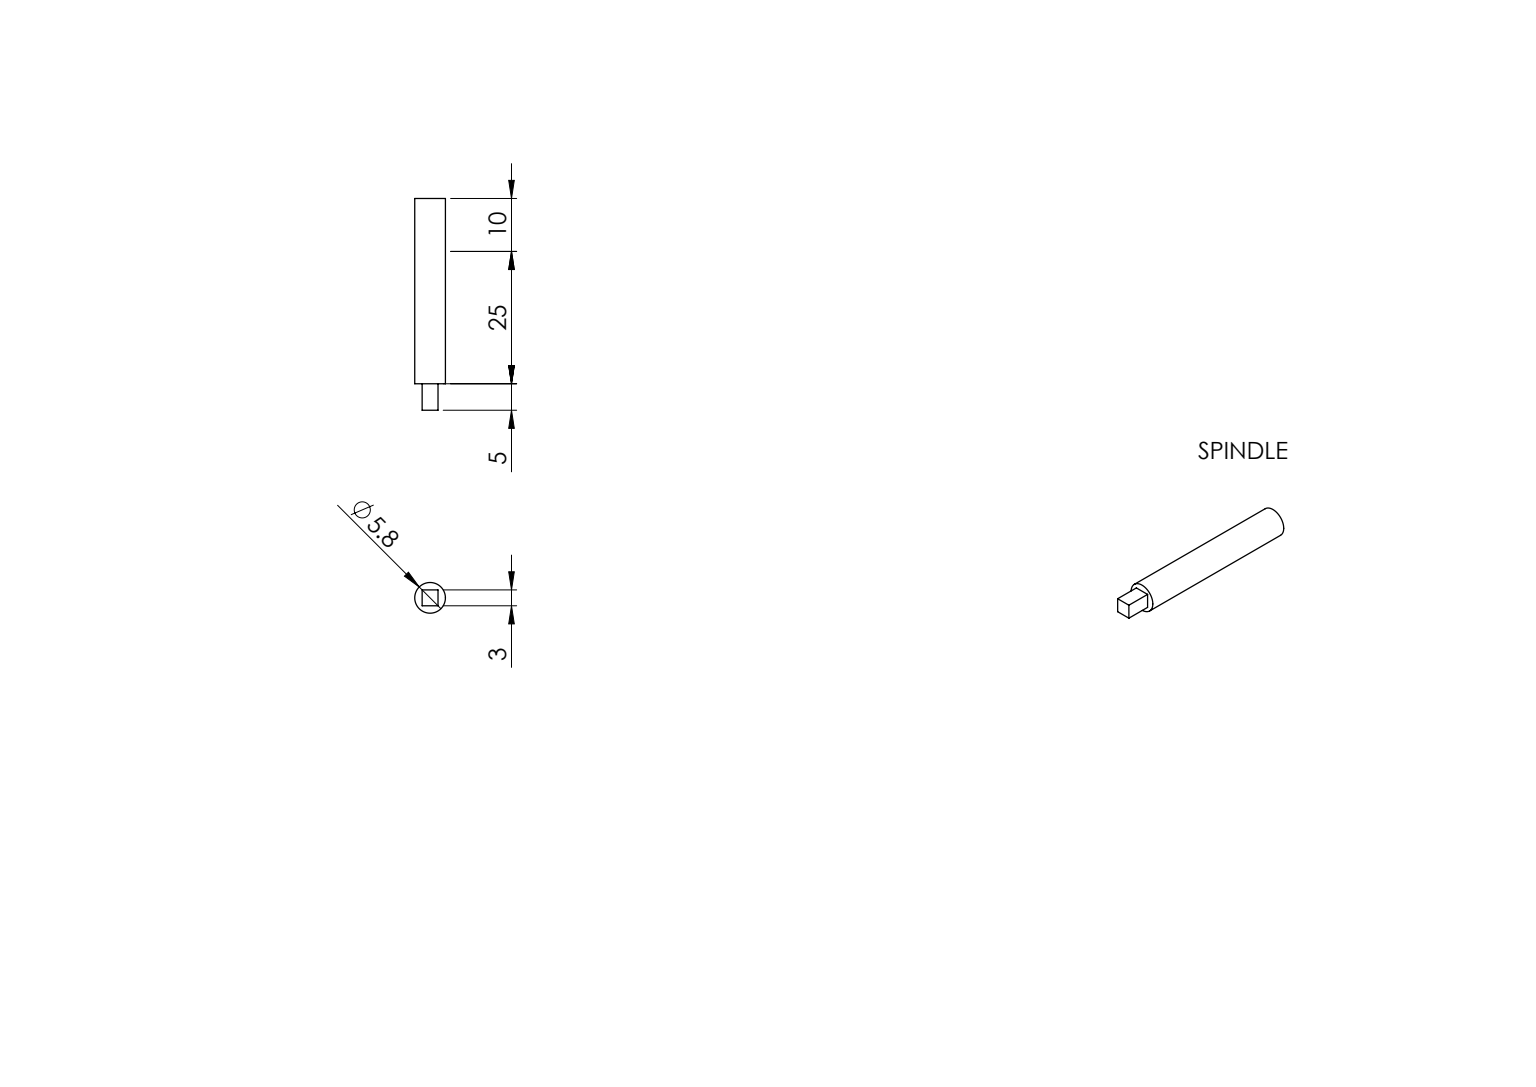
ISO-10303-21;
HEADER;
FILE_DESCRIPTION (('STEP AP214'),
    '1' );
FILE_NAME ('spindle.step',
    '2026-10-26T12:50:16',
    ( '' ),
    ( '' ),
    'SwSTEP 2.0',
    'SolidWorks 2026',
    '' );
FILE_SCHEMA (( 'AUTOMOTIVE_DESIGN' ));
ENDSEC;

DATA;
#229=PRODUCT_DEFINITION ( 'UNKNOWN', '', #18569, #2861 ) ;
#231=( LENGTH_UNIT ( ) NAMED_UNIT ( * ) SI_UNIT ( .MILLI., .METRE. ) );
#248=CARTESIAN_POINT ( 'NONE',  ( -2.899999999999996358, -8.999999999999992895, 25.00000000000000000 ) ) ;
#508=AXIS2_PLACEMENT_3D ( 'NONE', #23574, #21601, #11656 ) ;
#536=DIRECTION ( 'NONE',  ( -0.000000000000000000, -0.000000000000000000, -1.000000000000000000 ) ) ;
#569=( LENGTH_UNIT ( ) NAMED_UNIT ( * ) SI_UNIT ( .MILLI., .METRE. ) );
#621=CARTESIAN_POINT ( 'NONE',  ( 1.500000000000001776, -10.49999999999999289, 25.00000000000000000 ) ) ;
#636=PLANE ( 'NONE',  #20950 ) ;
#809=EDGE_CURVE ( 'NONE', #24918, #4288, #17286, .T. ) ;
#1026=ORIENTED_EDGE ( 'NONE', *, *, #13707, .T. ) ;
#1169=EDGE_CURVE ( 'NONE', #4288, #22996, #9088, .T. ) ;
#1252=PRODUCT_CONTEXT ( 'NONE', #12277, 'mechanical' ) ;
#1277=VERTEX_POINT ( 'NONE', #21768 ) ;
#1291=LINE ( 'NONE', #5217, #20952 ) ;
#1606=CARTESIAN_POINT ( 'NONE',  ( 2.900000000000003464, -8.999999999999992895, 25.00000000000000000 ) ) ;
#1677=CARTESIAN_POINT ( 'NONE',  ( -1.499999999999998224, -10.49999999999999289, 30.00000000000000355 ) ) ;
#2145=VERTEX_POINT ( 'NONE', #9561 ) ;
#2861=PRODUCT_DEFINITION_CONTEXT ( 'detailed design', #19293, 'design' ) ;
#2959=LINE ( 'NONE', #621, #13533 ) ;
#3022=EDGE_CURVE ( 'NONE', #11790, #1277, #20201, .T. ) ;
#3115=EDGE_LOOP ( 'NONE', ( #11167, #14069, #8642, #18079 ) ) ;
#3162=EDGE_CURVE ( 'NONE', #23707, #2145, #4900, .T. ) ;
#3167=ORIENTED_EDGE ( 'NONE', *, *, #10282, .F. ) ;
#3190=CARTESIAN_POINT ( 'NONE',  ( 3.469446951953614189E-15, -8.999999999999992895, -10.00000000000000000 ) ) ;
#3368=VECTOR ( 'NONE', #536, 1000.000000000000000 ) ;
#3395=AXIS2_PLACEMENT_3D ( 'NONE', #1677, #25474, #19072 ) ;
#3413=LINE ( 'NONE', #11515, #13794 ) ;
#3458=DIRECTION ( 'NONE',  ( -0.000000000000000000, -1.000000000000000000, -0.000000000000000000 ) ) ;
#3629=FACE_OUTER_BOUND ( 'NONE', #22399, .T. ) ;
#3707=ORIENTED_EDGE ( 'NONE', *, *, #13635, .T. ) ;
#3902=DIRECTION ( 'NONE',  ( 1.000000000000000000, -2.891205793294678326E-16, 0.000000000000000000 ) ) ;
#3928=CARTESIAN_POINT ( 'NONE',  ( 1.500000000000001776, -7.499999999999993783, 30.00000000000000355 ) ) ;
#3950=ORIENTED_EDGE ( 'NONE', *, *, #25431, .F. ) ;
#4149=PLANE ( 'NONE',  #7144 ) ;
#4224=EDGE_LOOP ( 'NONE', ( #11720, #19596, #3950, #3707 ) ) ;
#4277=FILL_AREA_STYLE ('',( #15786 ) ) ;
#4288=VERTEX_POINT ( 'NONE', #5621 ) ;
#4379=ORIENTED_EDGE ( 'NONE', *, *, #809, .T. ) ;
#4399=( NAMED_UNIT ( * ) PLANE_ANGLE_UNIT ( ) SI_UNIT ( $, .RADIAN. ) );
#4618=FACE_OUTER_BOUND ( 'NONE', #10624, .T. ) ;
#4787=LINE ( 'NONE', #12880, #22930 ) ;
#4900=LINE ( 'NONE', #11041, #15475 ) ;
#5075=ORIENTED_EDGE ( 'NONE', *, *, #1169, .T. ) ;
#5163=CARTESIAN_POINT ( 'NONE',  ( 3.469446951953614189E-15, -8.999999999999992895, 25.00000000000000000 ) ) ;
#5217=CARTESIAN_POINT ( 'NONE',  ( -2.899999999999996358, -8.999999999999992895, -10.00000000000000000 ) ) ;
#5280=DIRECTION ( 'NONE',  ( 1.000000000000000000, 0.000000000000000000, 0.000000000000000000 ) ) ;
#5338=DIRECTION ( 'NONE',  ( 1.000000000000000000, 0.000000000000000000, 0.000000000000000000 ) ) ;
#5380=CIRCLE ( 'NONE', #19982, 2.899999999999999911 ) ;
#5592=ORIENTED_EDGE ( 'NONE', *, *, #21469, .F. ) ;
#5621=CARTESIAN_POINT ( 'NONE',  ( 1.500000000000001776, -10.49999999999999289, 30.00000000000000355 ) ) ;
#5702=ORIENTED_EDGE ( 'NONE', *, *, #15200, .T. ) ;
#5767=EDGE_CURVE ( 'NONE', #2145, #11790, #2959, .T. ) ;
#5867=CARTESIAN_POINT ( 'NONE',  ( 1.500000000000001776, -10.49999999999999289, 30.00000000000000355 ) ) ;
#6229=SURFACE_SIDE_STYLE ('',( #18022 ) ) ;
#6292=ORIENTED_EDGE ( 'NONE', *, *, #21461, .T. ) ;
#6455=ADVANCED_FACE ( 'NONE', ( #17049 ), #17319, .F. ) ;
#6562=CARTESIAN_POINT ( 'NONE',  ( -1.499999999999998224, -7.499999999999992895, 30.00000000000000355 ) ) ;
#6818=ORIENTED_EDGE ( 'NONE', *, *, #18931, .F. ) ;
#6974=ADVANCED_FACE ( 'NONE', ( #22536, #4618 ), #10627, .T. ) ;
#6988=DIRECTION ( 'NONE',  ( 1.000000000000000000, -0.000000000000000000, -0.000000000000000000 ) ) ;
#7144=AXIS2_PLACEMENT_3D ( 'NONE', #12127, #20103, #10166 ) ;
#7146=CIRCLE ( 'NONE', #13012, 2.899999999999999911 ) ;
#7258=LINE ( 'NONE', #11039, #9168 ) ;
#7272=MECHANICAL_DESIGN_GEOMETRIC_PRESENTATION_REPRESENTATION('',(#22295),#10601);
#7376=CYLINDRICAL_SURFACE ( 'NONE', #19185, 2.899999999999999911 ) ;
#7419=CIRCLE ( 'NONE', #7887, 2.899999999999999911 ) ;
#7429=VERTEX_POINT ( 'NONE', #6562 ) ;
#7470=DIRECTION ( 'NONE',  ( 0.000000000000000000, 0.000000000000000000, 1.000000000000000000 ) ) ;
#7576=FACE_OUTER_BOUND ( 'NONE', #14240, .T. ) ;
#7676=( GEOMETRIC_REPRESENTATION_CONTEXT ( 3 ) GLOBAL_UNCERTAINTY_ASSIGNED_CONTEXT ( ( #10971 ) ) GLOBAL_UNIT_ASSIGNED_CONTEXT ( ( #231, #7808, #11863 ) ) REPRESENTATION_CONTEXT ( 'NONE', 'WORKASPACE' ) );
#7808=( NAMED_UNIT ( * ) PLANE_ANGLE_UNIT ( ) SI_UNIT ( $, .RADIAN. ) );
#7887=AXIS2_PLACEMENT_3D ( 'NONE', #5163, #13142, #5280 ) ;
#8126=FACE_OUTER_BOUND ( 'NONE', #17519, .T. ) ;
#8254=EDGE_CURVE ( 'NONE', #22773, #24763, #25592, .T. ) ;
#8445=ORIENTED_EDGE ( 'NONE', *, *, #13635, .F. ) ;
#8476=AXIS2_PLACEMENT_3D ( 'NONE', #22030, #24754, #23873 ) ;
#8531=ADVANCED_FACE ( 'NONE', ( #8126 ), #11787, .T. ) ;
#8642=ORIENTED_EDGE ( 'NONE', *, *, #15200, .F. ) ;
#8785=CARTESIAN_POINT ( 'NONE',  ( -2.899999999999996358, -8.999999999999992895, -10.00000000000000000 ) ) ;
#8843=CARTESIAN_POINT ( 'NONE',  ( 1.500000000000001776, -10.49999999999999289, 30.00000000000000355 ) ) ;
#8998=ORIENTED_EDGE ( 'NONE', *, *, #8254, .T. ) ;
#9061=VERTEX_POINT ( 'NONE', #248 ) ;
#9088=LINE ( 'NONE', #8843, #24740 ) ;
#9168=VECTOR ( 'NONE', #3458, 1000.000000000000000 ) ;
#9334=DIRECTION ( 'NONE',  ( -1.000000000000000000, 2.891205793294678326E-16, 0.000000000000000000 ) ) ;
#9561=CARTESIAN_POINT ( 'NONE',  ( 1.500000000000001776, -10.49999999999999289, 25.00000000000000000 ) ) ;
#9728=CARTESIAN_POINT ( 'NONE',  ( 2.900000000000003464, -8.999999999999992895, -10.00000000000000000 ) ) ;
#9760=ORIENTED_EDGE ( 'NONE', *, *, #21035, .T. ) ;
#9971=LINE ( 'NONE', #9728, #25848 ) ;
#10153=EDGE_CURVE ( 'NONE', #22773, #9061, #1291, .T. ) ;
#10166=DIRECTION ( 'NONE',  ( 0.000000000000000000, 0.000000000000000000, 1.000000000000000000 ) ) ;
#10177=ADVANCED_FACE ( 'NONE', ( #3629 ), #21429, .F. ) ;
#10258=DIRECTION ( 'NONE',  ( -1.000000000000000000, 2.891205793294678326E-16, 0.000000000000000000 ) ) ;
#10282=EDGE_CURVE ( 'NONE', #24763, #22773, #7146, .T. ) ;
#10491=AXIS2_PLACEMENT_3D ( 'NONE', #12859, #25020, #20837 ) ;
#10601=( GEOMETRIC_REPRESENTATION_CONTEXT ( 3 ) GLOBAL_UNCERTAINTY_ASSIGNED_CONTEXT ( ( #17261 ) ) GLOBAL_UNIT_ASSIGNED_CONTEXT ( ( #12116, #4399, #13832 ) ) REPRESENTATION_CONTEXT ( 'NONE', 'WORKASPACE' ) );
#10624=EDGE_LOOP ( 'NONE', ( #5702, #24649 ) ) ;
#10627=PLANE ( 'NONE',  #508 ) ;
#10948=ADVANCED_FACE ( 'NONE', ( #14097 ), #4149, .F. ) ;
#10971=UNCERTAINTY_MEASURE_WITH_UNIT (LENGTH_MEASURE( 1.000000000000000082E-05 ), #231, 'distance_accuracy_value', 'NONE');
#11039=CARTESIAN_POINT ( 'NONE',  ( -1.499999999999998224, -10.49999999999999289, 30.00000000000000355 ) ) ;
#11041=CARTESIAN_POINT ( 'NONE',  ( 1.500000000000001776, -10.49999999999999289, 25.00000000000000000 ) ) ;
#11167=ORIENTED_EDGE ( 'NONE', *, *, #10282, .T. ) ;
#11426=ORIENTED_EDGE ( 'NONE', *, *, #10153, .F. ) ;
#11515=CARTESIAN_POINT ( 'NONE',  ( 1.500000000000001776, -7.499999999999993783, 30.00000000000000355 ) ) ;
#11647=DIRECTION ( 'NONE',  ( 1.000000000000000000, 0.000000000000000000, 0.000000000000000000 ) ) ;
#11656=DIRECTION ( 'NONE',  ( 1.000000000000000000, 0.000000000000000000, -0.000000000000000000 ) ) ;
#11720=ORIENTED_EDGE ( 'NONE', *, *, #3022, .T. ) ;
#11787=CYLINDRICAL_SURFACE ( 'NONE', #18509, 2.899999999999999911 ) ;
#11790=VERTEX_POINT ( 'NONE', #11880 ) ;
#11843=ADVANCED_FACE ( 'NONE', ( #12663 ), #636, .T. ) ;
#11863=( NAMED_UNIT ( * ) SI_UNIT ( $, .STERADIAN. ) SOLID_ANGLE_UNIT ( ) );
#11880=CARTESIAN_POINT ( 'NONE',  ( 1.500000000000001776, -7.499999999999993783, 25.00000000000000000 ) ) ;
#12080=LINE ( 'NONE', #22290, #14598 ) ;
#12116=( LENGTH_UNIT ( ) NAMED_UNIT ( * ) SI_UNIT ( .MILLI., .METRE. ) );
#12126=CARTESIAN_POINT ( 'NONE',  ( 2.900000000000003464, -8.999999999999992895, -10.00000000000000000 ) ) ;
#12127=CARTESIAN_POINT ( 'NONE',  ( 1.500000000000001776, -10.49999999999999289, 30.00000000000000355 ) ) ;
#12252=PRESENTATION_STYLE_ASSIGNMENT (( #14085 ) ) ;
#12261=DIRECTION ( 'NONE',  ( -2.891205793294678326E-16, -1.000000000000000000, 0.000000000000000000 ) ) ;
#12277=APPLICATION_CONTEXT ( 'automotive_design' ) ;
#12376=SHAPE_REPRESENTATION_RELATIONSHIP ( 'NONE' , 'NONE' ,  #13517, #21253 ) ;
#12663=FACE_OUTER_BOUND ( 'NONE', #22952, .T. ) ;
#12750=CARTESIAN_POINT ( 'NONE',  ( 3.469446951953614189E-15, -8.999999999999992895, 25.00000000000000000 ) ) ;
#12859=CARTESIAN_POINT ( 'NONE',  ( 3.469446951953614189E-15, -8.999999999999992895, -10.00000000000000000 ) ) ;
#12880=CARTESIAN_POINT ( 'NONE',  ( -1.499999999999998224, -10.49999999999999289, 25.00000000000000000 ) ) ;
#12983=CLOSED_SHELL ( 'NONE', ( #20116, #8531, #6455, #6974, #10177, #10948, #17461, #24835, #11843 ) ) ;
#13012=AXIS2_PLACEMENT_3D ( 'NONE', #21050, #13462, #5338 ) ;
#13083=VECTOR ( 'NONE', #9334, 1000.000000000000000 ) ;
#13142=DIRECTION ( 'NONE',  ( 0.000000000000000000, 0.000000000000000000, 1.000000000000000000 ) ) ;
#13223=DIRECTION ( 'NONE',  ( 1.000000000000000000, 0.000000000000000000, 0.000000000000000000 ) ) ;
#13271=MANIFOLD_SOLID_BREP ( 'Boss-Extrude2', #12983 ) ;
#13346=CARTESIAN_POINT ( 'NONE',  ( 1.500000000000001776, -10.49999999999999289, 30.00000000000000355 ) ) ;
#13353=CARTESIAN_POINT ( 'NONE',  ( 0.000000000000000000, 0.000000000000000000, 0.000000000000000000 ) ) ;
#13373=ORIENTED_EDGE ( 'NONE', *, *, #19950, .T. ) ;
#13462=DIRECTION ( 'NONE',  ( 0.000000000000000000, 0.000000000000000000, 1.000000000000000000 ) ) ;
#13517=SHAPE_REPRESENTATION ( 'spindle', ( #21036 ), #7676 ) ;
#13533=VECTOR ( 'NONE', #18650, 1000.000000000000000 ) ;
#13635=EDGE_CURVE ( 'NONE', #22996, #11790, #3413, .T. ) ;
#13707=EDGE_CURVE ( 'NONE', #7429, #1277, #22091, .T. ) ;
#13794=VECTOR ( 'NONE', #17539, 1000.000000000000000 ) ;
#13832=( NAMED_UNIT ( * ) SI_UNIT ( $, .STERADIAN. ) SOLID_ANGLE_UNIT ( ) );
#13851=DIRECTION ( 'NONE',  ( -1.000000000000000000, 0.000000000000000000, 0.000000000000000000 ) ) ;
#13856=EDGE_LOOP ( 'NONE', ( #25418, #17554, #23441, #18388 ) ) ;
#14012=CARTESIAN_POINT ( 'NONE',  ( 3.469446951953614189E-15, -8.999999999999992895, -10.00000000000000000 ) ) ;
#14056=DIRECTION ( 'NONE',  ( -0.000000000000000000, -0.000000000000000000, -1.000000000000000000 ) ) ;
#14069=ORIENTED_EDGE ( 'NONE', *, *, #10153, .T. ) ;
#14085=SURFACE_STYLE_USAGE ( .BOTH. , #6229 ) ;
#14097=FACE_OUTER_BOUND ( 'NONE', #19474, .T. ) ;
#14240=EDGE_LOOP ( 'NONE', ( #17690, #8445, #17476, #6292 ) ) ;
#14396=CARTESIAN_POINT ( 'NONE',  ( -1.499999999999998224, -7.499999999999992895, 30.00000000000000355 ) ) ;
#14411=ORIENTED_EDGE ( 'NONE', *, *, #21469, .T. ) ;
#14450=LINE ( 'NONE', #23991, #24620 ) ;
#14555=ORIENTED_EDGE ( 'NONE', *, *, #3162, .T. ) ;
#14598=VECTOR ( 'NONE', #14056, 1000.000000000000000 ) ;
#14661=ORIENTED_EDGE ( 'NONE', *, *, #8254, .F. ) ;
#15200=EDGE_CURVE ( 'NONE', #21831, #9061, #7419, .T. ) ;
#15311=EDGE_CURVE ( 'NONE', #24763, #21831, #9971, .T. ) ;
#15475=VECTOR ( 'NONE', #6988, 1000.000000000000000 ) ;
#15548=DIRECTION ( 'NONE',  ( 0.000000000000000000, 0.000000000000000000, 1.000000000000000000 ) ) ;
#15703=DIRECTION ( 'NONE',  ( 0.000000000000000000, 0.000000000000000000, 1.000000000000000000 ) ) ;
#15741=DIRECTION ( 'NONE',  ( 0.000000000000000000, 0.000000000000000000, 1.000000000000000000 ) ) ;
#15786=FILL_AREA_STYLE_COLOUR ( '', #18551 ) ;
#16121=PRODUCT_DEFINITION_SHAPE ( 'NONE', 'NONE',  #229 ) ;
#16546=VECTOR ( 'NONE', #19219, 1000.000000000000000 ) ;
#16683=DIRECTION ( 'NONE',  ( -0.000000000000000000, -1.000000000000000000, -0.000000000000000000 ) ) ;
#16687=DIRECTION ( 'NONE',  ( 0.000000000000000000, 1.000000000000000000, 0.000000000000000000 ) ) ;
#17049=FACE_OUTER_BOUND ( 'NONE', #24885, .T. ) ;
#17104=AXIS2_PLACEMENT_3D ( 'NONE', #5867, #13851, #19972 ) ;
#17261=UNCERTAINTY_MEASURE_WITH_UNIT (LENGTH_MEASURE( 1.000000000000000082E-05 ), #12116, 'distance_accuracy_value', 'NONE');
#17286=LINE ( 'NONE', #13346, #16546 ) ;
#17319=PLANE ( 'NONE',  #10491 ) ;
#17461=ADVANCED_FACE ( 'NONE', ( #7576 ), #19734, .F. ) ;
#17476=ORIENTED_EDGE ( 'NONE', *, *, #1169, .F. ) ;
#17519=EDGE_LOOP ( 'NONE', ( #11426, #8998, #18468, #6818 ) ) ;
#17539=DIRECTION ( 'NONE',  ( -0.000000000000000000, -0.000000000000000000, -1.000000000000000000 ) ) ;
#17554=ORIENTED_EDGE ( 'NONE', *, *, #3022, .F. ) ;
#17690=ORIENTED_EDGE ( 'NONE', *, *, #5767, .T. ) ;
#17927=DIRECTION ( 'NONE',  ( 0.000000000000000000, 0.000000000000000000, 1.000000000000000000 ) ) ;
#18022=SURFACE_STYLE_FILL_AREA ( #4277 ) ;
#18079=ORIENTED_EDGE ( 'NONE', *, *, #15311, .F. ) ;
#18388=ORIENTED_EDGE ( 'NONE', *, *, #3162, .F. ) ;
#18468=ORIENTED_EDGE ( 'NONE', *, *, #15311, .T. ) ;
#18509=AXIS2_PLACEMENT_3D ( 'NONE', #14012, #17927, #11647 ) ;
#18546=CARTESIAN_POINT ( 'NONE',  ( -1.499999999999998224, -10.49999999999999289, 30.00000000000000355 ) ) ;
#18551=COLOUR_RGB ( '',0.8941176470588234615, 0.8941176470588234615, 0.8941176470588234615 ) ;
#18569=PRODUCT_DEFINITION_FORMATION_WITH_SPECIFIED_SOURCE ( 'ANY', '', #20064, .NOT_KNOWN. ) ;
#18650=DIRECTION ( 'NONE',  ( 0.000000000000000000, 1.000000000000000000, 0.000000000000000000 ) ) ;
#18769=ORIENTED_EDGE ( 'NONE', *, *, #19950, .F. ) ;
#18902=FACE_OUTER_BOUND ( 'NONE', #3115, .T. ) ;
#18931=EDGE_CURVE ( 'NONE', #9061, #21831, #5380, .T. ) ;
#18940=ORIENTED_EDGE ( 'NONE', *, *, #21461, .F. ) ;
#19072=DIRECTION ( 'NONE',  ( 0.000000000000000000, 0.000000000000000000, -1.000000000000000000 ) ) ;
#19185=AXIS2_PLACEMENT_3D ( 'NONE', #3190, #23324, #21378 ) ;
#19219=DIRECTION ( 'NONE',  ( 1.000000000000000000, -0.000000000000000000, -0.000000000000000000 ) ) ;
#19293=APPLICATION_CONTEXT ( 'automotive_design' ) ;
#19474=EDGE_LOOP ( 'NONE', ( #14555, #18940, #23299, #14411 ) ) ;
#19596=ORIENTED_EDGE ( 'NONE', *, *, #13707, .F. ) ;
#19620=VECTOR ( 'NONE', #10258, 1000.000000000000000 ) ;
#19734=PLANE ( 'NONE',  #17104 ) ;
#19840=FACE_OUTER_BOUND ( 'NONE', #4224, .T. ) ;
#19950=EDGE_CURVE ( 'NONE', #7429, #24918, #7258, .T. ) ;
#19972=DIRECTION ( 'NONE',  ( 0.000000000000000000, 0.000000000000000000, 1.000000000000000000 ) ) ;
#19982=AXIS2_PLACEMENT_3D ( 'NONE', #12750, #7470, #20721 ) ;
#20016=STYLED_ITEM('',(#25907),#13271);
#20064=PRODUCT ( 'spindle', 'spindle', '', ( #1252 ) ) ;
#20103=DIRECTION ( 'NONE',  ( 0.000000000000000000, 1.000000000000000000, -0.000000000000000000 ) ) ;
#20116=ADVANCED_FACE ( 'NONE', ( #18902 ), #7376, .T. ) ;
#20201=LINE ( 'NONE', #20326, #19620 ) ;
#20326=CARTESIAN_POINT ( 'NONE',  ( 1.500000000000001776, -7.499999999999993783, 25.00000000000000000 ) ) ;
#20349=PLANE ( 'NONE',  #21808 ) ;
#20480=CARTESIAN_POINT ( 'NONE',  ( -1.499999999999998224, -10.49999999999999289, 25.00000000000000000 ) ) ;
#20721=DIRECTION ( 'NONE',  ( 1.000000000000000000, 0.000000000000000000, 0.000000000000000000 ) ) ;
#20760=DIRECTION ( 'NONE',  ( 1.000000000000000000, 0.000000000000000000, -0.000000000000000000 ) ) ;
#20837=DIRECTION ( 'NONE',  ( 1.000000000000000000, 0.000000000000000000, -0.000000000000000000 ) ) ;
#20950=AXIS2_PLACEMENT_3D ( 'NONE', #21028, #24686, #20760 ) ;
#20952=VECTOR ( 'NONE', #15548, 1000.000000000000000 ) ;
#21028=CARTESIAN_POINT ( 'NONE',  ( 0.000000000000000000, 0.000000000000000000, 30.00000000000000355 ) ) ;
#21035=EDGE_CURVE ( 'NONE', #1277, #23707, #4787, .T. ) ;
#21036=AXIS2_PLACEMENT_3D ( 'NONE', #13353, #15703, #13223 ) ;
#21050=CARTESIAN_POINT ( 'NONE',  ( 3.469446951953614189E-15, -8.999999999999992895, -10.00000000000000000 ) ) ;
#21253=ADVANCED_BREP_SHAPE_REPRESENTATION ( '', ( #13271, #21036 ), #7676 ) ;
#21378=DIRECTION ( 'NONE',  ( 1.000000000000000000, 0.000000000000000000, 0.000000000000000000 ) ) ;
#21429=PLANE ( 'NONE',  #3395 ) ;
#21461=EDGE_CURVE ( 'NONE', #4288, #2145, #12080, .T. ) ;
#21469=EDGE_CURVE ( 'NONE', #24918, #23707, #14450, .T. ) ;
#21488=LINE ( 'NONE', #23443, #13083 ) ;
#21601=DIRECTION ( 'NONE',  ( 0.000000000000000000, 0.000000000000000000, 1.000000000000000000 ) ) ;
#21768=CARTESIAN_POINT ( 'NONE',  ( -1.499999999999998224, -7.499999999999992895, 25.00000000000000000 ) ) ;
#21776=( NAMED_UNIT ( * ) SI_UNIT ( $, .STERADIAN. ) SOLID_ANGLE_UNIT ( ) );
#21808=AXIS2_PLACEMENT_3D ( 'NONE', #22202, #12261, #3902 ) ;
#21831=VERTEX_POINT ( 'NONE', #1606 ) ;
#21867=ORIENTED_EDGE ( 'NONE', *, *, #25431, .T. ) ;
#22022=DIRECTION ( 'NONE',  ( -0.000000000000000000, -0.000000000000000000, -1.000000000000000000 ) ) ;
#22025=( NAMED_UNIT ( * ) PLANE_ANGLE_UNIT ( ) SI_UNIT ( $, .RADIAN. ) );
#22030=CARTESIAN_POINT ( 'NONE',  ( 3.469446951953614189E-15, -8.999999999999992895, -10.00000000000000000 ) ) ;
#22091=LINE ( 'NONE', #14396, #3368 ) ;
#22131=MECHANICAL_DESIGN_GEOMETRIC_PRESENTATION_REPRESENTATION('',(#20016),#24630);
#22202=CARTESIAN_POINT ( 'NONE',  ( 1.500000000000001776, -7.499999999999993783, 30.00000000000000355 ) ) ;
#22290=CARTESIAN_POINT ( 'NONE',  ( 1.500000000000001776, -10.49999999999999289, 30.00000000000000355 ) ) ;
#22295=STYLED_ITEM ( 'NONE', ( #12252 ), #21253 ) ;
#22399=EDGE_LOOP ( 'NONE', ( #9760, #5592, #18769, #1026 ) ) ;
#22536=FACE_BOUND ( 'NONE', #13856, .T. ) ;
#22773=VERTEX_POINT ( 'NONE', #8785 ) ;
#22930=VECTOR ( 'NONE', #16683, 1000.000000000000000 ) ;
#22952=EDGE_LOOP ( 'NONE', ( #13373, #4379, #5075, #21867 ) ) ;
#22996=VERTEX_POINT ( 'NONE', #3928 ) ;
#23103=SHAPE_DEFINITION_REPRESENTATION ( #16121, #13517 ) ;
#23299=ORIENTED_EDGE ( 'NONE', *, *, #809, .F. ) ;
#23324=DIRECTION ( 'NONE',  ( 0.000000000000000000, 0.000000000000000000, 1.000000000000000000 ) ) ;
#23441=ORIENTED_EDGE ( 'NONE', *, *, #5767, .F. ) ;
#23443=CARTESIAN_POINT ( 'NONE',  ( 1.500000000000001776, -7.499999999999993783, 30.00000000000000355 ) ) ;
#23574=CARTESIAN_POINT ( 'NONE',  ( 3.469446951953614189E-15, -8.999999999999992895, 25.00000000000000000 ) ) ;
#23707=VERTEX_POINT ( 'NONE', #20480 ) ;
#23873=DIRECTION ( 'NONE',  ( 1.000000000000000000, 0.000000000000000000, 0.000000000000000000 ) ) ;
#23991=CARTESIAN_POINT ( 'NONE',  ( -1.499999999999998224, -10.49999999999999289, 30.00000000000000355 ) ) ;
#24566=UNCERTAINTY_MEASURE_WITH_UNIT (LENGTH_MEASURE( 1.000000000000000082E-05 ), #569, 'distance_accuracy_value', 'NONE');
#24620=VECTOR ( 'NONE', #22022, 1000.000000000000000 ) ;
#24630=( GEOMETRIC_REPRESENTATION_CONTEXT ( 3 ) GLOBAL_UNCERTAINTY_ASSIGNED_CONTEXT ( ( #24566 ) ) GLOBAL_UNIT_ASSIGNED_CONTEXT ( ( #569, #22025, #21776 ) ) REPRESENTATION_CONTEXT ( 'NONE', 'WORKASPACE' ) );
#24649=ORIENTED_EDGE ( 'NONE', *, *, #18931, .T. ) ;
#24686=DIRECTION ( 'NONE',  ( 0.000000000000000000, -0.000000000000000000, 1.000000000000000000 ) ) ;
#24740=VECTOR ( 'NONE', #16687, 1000.000000000000000 ) ;
#24754=DIRECTION ( 'NONE',  ( 0.000000000000000000, 0.000000000000000000, 1.000000000000000000 ) ) ;
#24763=VERTEX_POINT ( 'NONE', #12126 ) ;
#24835=ADVANCED_FACE ( 'NONE', ( #19840 ), #20349, .F. ) ;
#24885=EDGE_LOOP ( 'NONE', ( #3167, #14661 ) ) ;
#24918=VERTEX_POINT ( 'NONE', #18546 ) ;
#25020=DIRECTION ( 'NONE',  ( 0.000000000000000000, 0.000000000000000000, 1.000000000000000000 ) ) ;
#25418=ORIENTED_EDGE ( 'NONE', *, *, #21035, .F. ) ;
#25431=EDGE_CURVE ( 'NONE', #22996, #7429, #21488, .T. ) ;
#25474=DIRECTION ( 'NONE',  ( 1.000000000000000000, 0.000000000000000000, 0.000000000000000000 ) ) ;
#25592=CIRCLE ( 'NONE', #8476, 2.899999999999999911 ) ;
#25848=VECTOR ( 'NONE', #15741, 1000.000000000000000 ) ;
#25901=COLOUR_RGB('Sky Blue',0.24,0.69,0.87);
#25902=FILL_AREA_STYLE_COLOUR('',#25901);
#25903=FILL_AREA_STYLE('',(#25902));
#25904=SURFACE_STYLE_FILL_AREA(#25903);
#25905=SURFACE_SIDE_STYLE('',(#25904));
#25906=SURFACE_STYLE_USAGE(.BOTH.,#25905);
#25907=PRESENTATION_STYLE_ASSIGNMENT((#25906));
ENDSEC;
END-ISO-10303-21;
